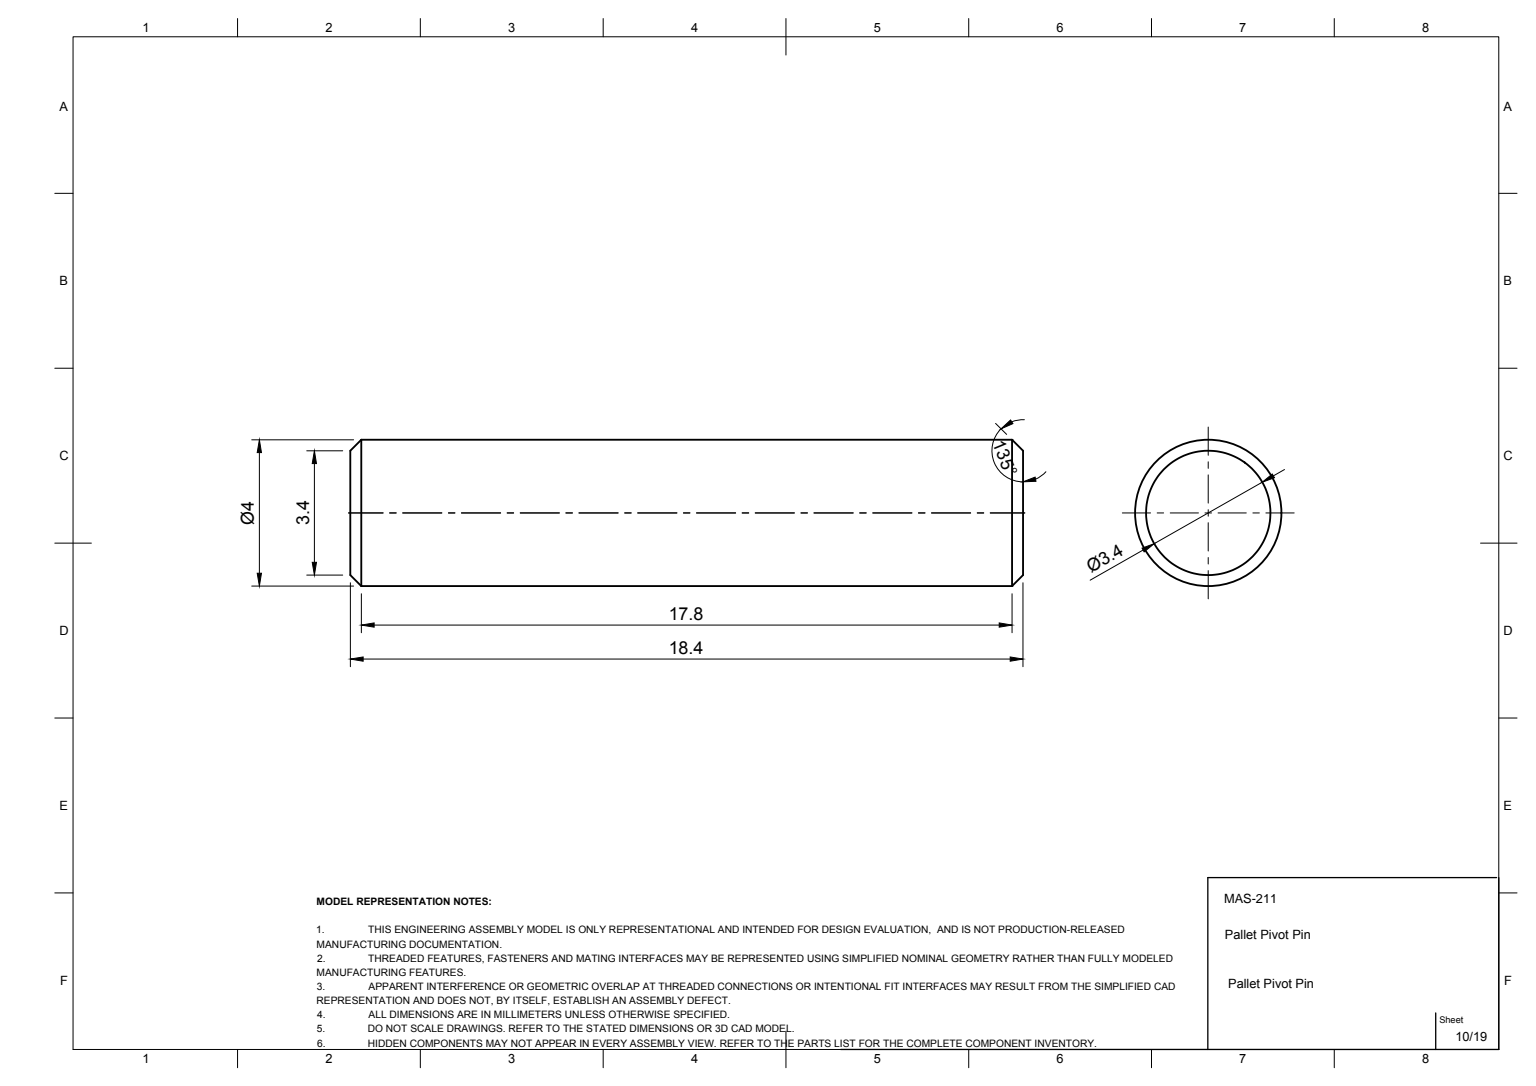
ISO-10303-21;
HEADER;
FILE_DESCRIPTION(
 (''),
 '2;1');
FILE_NAME ( 'Pallet Pivot Pin.step', '2026-10-05T20:07:59+06:00', ( '' ), ( '' ), 'STEP AP214', 'Unspecified', '' );
FILE_SCHEMA (('AUTOMOTIVE_DESIGN { 1 0 10303 214 3 1 1 }'));
ENDSEC;
DATA;
#10=MECHANICAL_DESIGN_GEOMETRIC_PRESENTATION_REPRESENTATION('',(#327),#196741);
#327=STYLED_ITEM('',(#196765),#346) ;
#346=MANIFOLD_SOLID_BREP('Pallet Pivot Pin',#8723) ;
#389=PLANE('',#8938) ;
#390=PLANE('',#8939) ;
#687=CIRCLE('',#8936,2.00000000000002) ;
#688=CIRCLE('',#8937,2.00000000000002) ;
#857=B_SPLINE_SURFACE_WITH_KNOTS('',1,3,((#113835,#113836,#113837,#113838,
#113839,#113840,#113841,#113842,#113843,#113844,#113845,#113846,#113847,
#113848,#113849,#113850,#113851,#113852,#113853),(#113854,#113855,#113856,
#113857,#113858,#113859,#113860,#113861,#113862,#113863,#113864,#113865,
#113866,#113867,#113868,#113869,#113870,#113871,#113872)),.UNSPECIFIED.,
 .F.,.T.,.F.,(2,2),(4,1,1,1,1,1,1,1,1,1,1,1,1,1,1,1,4),(0.,0.431146952730274),
(0.,0.667571568814079,1.33514313762816,2.00271471386765,2.67028629010715,
3.33785785892125,4.00542942773535,4.67300100397484,5.34057258021434,6.00814415645112,
6.67571573268789,7.34328730150198,8.01085887031606,8.67843044655556,9.34600202279505,
10.0135735916092,10.6811451604233),.UNSPECIFIED.) ;
#858=B_SPLINE_SURFACE_WITH_KNOTS('',3,1,((#113874,#113875),(#113876,#113877),
(#113878,#113879),(#113880,#113881),(#113882,#113883),(#113884,#113885),
(#113886,#113887),(#113888,#113889),(#113890,#113891),(#113892,#113893),
(#113894,#113895),(#113896,#113897),(#113898,#113899),(#113900,#113901),
(#113902,#113903),(#113904,#113905),(#113906,#113907),(#113908,#113909),
(#113910,#113911)),.UNSPECIFIED.,.T.,.F.,.F.,(4,1,1,1,1,1,1,1,1,1,1,1,1,
1,1,1,4),(2,2),(0.,0.667571568814083,1.33514313762817,2.00271471386766,
2.67028629010715,3.33785785892125,4.00542942773535,4.67300100397484,5.34057258021433,
6.00814415645111,6.67571573268789,7.34328730150198,8.01085887031607,8.67843044655557,
9.34600202279507,10.0135735916092,10.6811451604233),(0.,0.431146952730387),
 .UNSPECIFIED.) ;
#1009=FACE_OUTER_BOUND('',#1514,.T.) ;
#1010=FACE_OUTER_BOUND('',#1515,.T.) ;
#1011=FACE_OUTER_BOUND('',#1516,.T.) ;
#1012=FACE_OUTER_BOUND('',#1517,.T.) ;
#1013=FACE_OUTER_BOUND('',#1518,.T.) ;
#1514=EDGE_LOOP('',(#6350,#6351,#6352,#6353)) ;
#1515=EDGE_LOOP('',(#6354)) ;
#1516=EDGE_LOOP('',(#6355)) ;
#1517=EDGE_LOOP('',(#6356,#6357,#6358,#6359)) ;
#1518=EDGE_LOOP('',(#6360,#6361,#6362,#6363)) ;
#2007=LINE('',#113791,#2710) ;
#2008=LINE('',#113873,#2711) ;
#2009=LINE('',#113912,#2712) ;
#2710=VECTOR('',#9981,2.00000000000003) ;
#2711=VECTOR('',#9988,10.) ;
#2712=VECTOR('',#9989,10.) ;
#3433=B_SPLINE_CURVE_WITH_KNOTS('',3,(#113795,#113796,#113797,#113798,#113799,
#113800,#113801,#113802,#113803,#113804,#113805,#113806,#113807,#113808,
#113809,#113810,#113811,#113812,#113813),.UNSPECIFIED.,.T.,.F.,(4,1,1,1,
1,1,1,1,1,1,1,1,1,1,1,1,4),(0.,0.667571568814079,1.33514313762816,2.00271471386765,
2.67028629010715,3.33785785892125,4.00542942773535,4.67300100397484,5.34057258021434,
6.00814415645112,6.67571573268789,7.34328730150198,8.01085887031606,8.67843044655556,
9.34600202279505,10.0135735916092,10.6811451604233),.UNSPECIFIED.) ;
#3434=B_SPLINE_CURVE_WITH_KNOTS('',3,(#113816,#113817,#113818,#113819,#113820,
#113821,#113822,#113823,#113824,#113825,#113826,#113827,#113828,#113829,
#113830,#113831,#113832,#113833,#113834),.UNSPECIFIED.,.T.,.F.,(4,1,1,1,
1,1,1,1,1,1,1,1,1,1,1,1,4),(0.,0.667571568814083,1.33514313762817,2.00271471386766,
2.67028629010715,3.33785785892125,4.00542942773535,4.67300100397484,5.34057258021433,
6.00814415645111,6.67571573268789,7.34328730150198,8.01085887031607,8.67843044655557,
9.34600202279507,10.0135735916092,10.6811451604233),.UNSPECIFIED.) ;
#3704=VERTEX_POINT('',#113788) ;
#3705=VERTEX_POINT('',#113790) ;
#3706=VERTEX_POINT('',#113794) ;
#3707=VERTEX_POINT('',#113815) ;
#4683=EDGE_CURVE('',#3704,#3704,#687,.T.) ;
#4684=EDGE_CURVE('',#3704,#3705,#2007,.T.) ;
#4685=EDGE_CURVE('',#3705,#3705,#688,.T.) ;
#4686=EDGE_CURVE('',#3706,#3706,#3433,.T.) ;
#4687=EDGE_CURVE('',#3707,#3707,#3434,.T.) ;
#4688=EDGE_CURVE('',#3704,#3706,#2008,.T.) ;
#4689=EDGE_CURVE('',#3705,#3707,#2009,.T.) ;
#6350=ORIENTED_EDGE('',*,*,#4683,.T.) ;
#6351=ORIENTED_EDGE('',*,*,#4684,.T.) ;
#6352=ORIENTED_EDGE('',*,*,#4685,.F.) ;
#6353=ORIENTED_EDGE('',*,*,#4684,.F.) ;
#6354=ORIENTED_EDGE('',*,*,#4686,.F.) ;
#6355=ORIENTED_EDGE('',*,*,#4687,.T.) ;
#6356=ORIENTED_EDGE('',*,*,#4688,.T.) ;
#6357=ORIENTED_EDGE('',*,*,#4686,.T.) ;
#6358=ORIENTED_EDGE('',*,*,#4688,.F.) ;
#6359=ORIENTED_EDGE('',*,*,#4683,.F.) ;
#6360=ORIENTED_EDGE('',*,*,#4685,.T.) ;
#6361=ORIENTED_EDGE('',*,*,#4689,.T.) ;
#6362=ORIENTED_EDGE('',*,*,#4687,.F.) ;
#6363=ORIENTED_EDGE('',*,*,#4689,.F.) ;
#8184=CYLINDRICAL_SURFACE('',#8935,2.00000000000003) ;
#8392=ADVANCED_FACE('',(#1009),#8184,.T.) ;
#8393=ADVANCED_FACE('',(#1010),#389,.T.) ;
#8394=ADVANCED_FACE('',(#1011),#390,.T.) ;
#8395=ADVANCED_FACE('',(#1012),#857,.T.) ;
#8396=ADVANCED_FACE('',(#1013),#858,.T.) ;
#8723=CLOSED_SHELL('',(#8392,#8393,#8394,#8395,#8396)) ;
#8935=AXIS2_PLACEMENT_3D('',#113787,#9977,#9978) ;
#8936=AXIS2_PLACEMENT_3D('',#113789,#9979,#9980) ;
#8937=AXIS2_PLACEMENT_3D('',#113792,#9982,#9983) ;
#8938=AXIS2_PLACEMENT_3D('',#113793,#9984,#9985) ;
#8939=AXIS2_PLACEMENT_3D('',#113814,#9986,#9987) ;
#9977=DIRECTION('center_axis',(0.,-1.,0.)) ;
#9978=DIRECTION('ref_axis',(0.587391769794684,0.,-0.809302729995068)) ;
#9979=DIRECTION('center_axis',(-6.57177564856263E-16,1.,-6.46151479728032E-16)) ;
#9980=DIRECTION('ref_axis',(-0.948327476740895,-5.55111512312572E-16,0.317293234813235)) ;
#9981=DIRECTION('',(0.,1.,0.)) ;
#9982=DIRECTION('center_axis',(1.11571400579693E-15,1.,3.09771438098241E-16)) ;
#9983=DIRECTION('ref_axis',(-0.948327476740895,1.11022302462514E-15,0.317293234813235)) ;
#9984=DIRECTION('center_axis',(0.,-1.,0.)) ;
#9985=DIRECTION('ref_axis',(0.,0.,-1.)) ;
#9986=DIRECTION('center_axis',(0.,1.,0.)) ;
#9987=DIRECTION('ref_axis',(0.,0.,1.)) ;
#9988=DIRECTION('',(0.415348703634992,-0.707106781186545,-0.572263448412299)) ;
#9989=DIRECTION('',(0.415348703634974,0.707106781186551,-0.572263448412304)) ;
#113787=CARTESIAN_POINT('Origin',(-28.8703041205685,-9.2000000000496,120.173187866852)) ;
#113788=CARTESIAN_POINT('',(-30.0450876601579,-8.90000000004959,121.791793326842)) ;
#113789=CARTESIAN_POINT('Origin',(-28.8703041205685,-8.90000000004959,120.173187866852)) ;
#113790=CARTESIAN_POINT('',(-30.0450876601579,8.90000000004959,121.791793326842)) ;
#113791=CARTESIAN_POINT('',(-30.0450876601579,-9.2000000000496,121.791793326842)) ;
#113792=CARTESIAN_POINT('Origin',(-28.8703041205685,8.90000000004959,120.173187866852)) ;
#113793=CARTESIAN_POINT('Origin',(-30.0450876601579,-9.2000000000496,121.791793326842)) ;
#113794=CARTESIAN_POINT('',(-29.8688701292195,-9.2000000000496,121.549002507844)) ;
#113795=CARTESIAN_POINT('Ctrl Pts',(-29.8688701292195,-9.2000000000496,
121.549002507844)) ;
#113796=CARTESIAN_POINT('Ctrl Pts',(-29.6888722586779,-9.2000000000496,
121.679801257268)) ;
#113797=CARTESIAN_POINT('Ctrl Pts',(-29.2766671363574,-9.2000000000496,
121.869462570365)) ;
#113798=CARTESIAN_POINT('Ctrl Pts',(-28.5966094899589,-9.20000000004961,
121.895918474133)) ;
#113799=CARTESIAN_POINT('Ctrl Pts',(-27.9581738536376,-9.20000000004958,
121.660008974116)) ;
#113800=CARTESIAN_POINT('Ctrl Pts',(-27.4586313028868,-9.20000000004961,
121.197792875516)) ;
#113801=CARTESIAN_POINT('Ctrl Pts',(-27.1739845654614,-9.20000000004959,
120.579569231899)) ;
#113802=CARTESIAN_POINT('Ctrl Pts',(-27.1475967294287,-9.2000000000496,
119.899485204542)) ;
#113803=CARTESIAN_POINT('Ctrl Pts',(-27.3834704179729,-9.20000000004961,
119.261061767752)) ;
#113804=CARTESIAN_POINT('Ctrl Pts',(-27.8457060572027,-9.20000000004959,
118.761512772263)) ;
#113805=CARTESIAN_POINT('Ctrl Pts',(-28.4639187630298,-9.20000000004959,
118.476869616603)) ;
#113806=CARTESIAN_POINT('Ctrl Pts',(-29.1440090539224,-9.2000000000496,
118.450479738512)) ;
#113807=CARTESIAN_POINT('Ctrl Pts',(-29.7824289744744,-9.20000000004958,
118.686354577768)) ;
#113808=CARTESIAN_POINT('Ctrl Pts',(-30.2819799090915,-9.2000000000496,
119.148589579807)) ;
#113809=CARTESIAN_POINT('Ctrl Pts',(-30.5666217872644,-9.2000000000496,
119.766803935434)) ;
#113810=CARTESIAN_POINT('Ctrl Pts',(-30.593025972774,-9.20000000004959,
120.446909151552)) ;
#113811=CARTESIAN_POINT('Ctrl Pts',(-30.3571041737437,-9.2000000000496,
121.085287178393)) ;
#113812=CARTESIAN_POINT('Ctrl Pts',(-30.0490282665823,-9.20000000004959,
121.418401787627)) ;
#113813=CARTESIAN_POINT('Ctrl Pts',(-29.8688701292195,-9.2000000000496,
121.549002507844)) ;
#113814=CARTESIAN_POINT('Origin',(-30.0450876601579,9.2000000000496,121.791793326842)) ;
#113815=CARTESIAN_POINT('',(-29.8688701292195,9.2000000000496,121.549002507844)) ;
#113816=CARTESIAN_POINT('Ctrl Pts',(-29.8688701292195,9.2000000000496,121.549002507844)) ;
#113817=CARTESIAN_POINT('Ctrl Pts',(-29.6888722586779,9.2000000000496,121.679801257268)) ;
#113818=CARTESIAN_POINT('Ctrl Pts',(-29.2766671363573,9.20000000004959,
121.869462570365)) ;
#113819=CARTESIAN_POINT('Ctrl Pts',(-28.5966094899589,9.20000000004961,
121.895918474133)) ;
#113820=CARTESIAN_POINT('Ctrl Pts',(-27.9581738536375,9.20000000004957,
121.660008974116)) ;
#113821=CARTESIAN_POINT('Ctrl Pts',(-27.4586313028868,9.20000000004962,
121.197792875516)) ;
#113822=CARTESIAN_POINT('Ctrl Pts',(-27.1739845654613,9.20000000004957,
120.579569231898)) ;
#113823=CARTESIAN_POINT('Ctrl Pts',(-27.1475967294288,9.20000000004963,
119.899485204542)) ;
#113824=CARTESIAN_POINT('Ctrl Pts',(-27.3834704179728,9.20000000004958,
119.261061767752)) ;
#113825=CARTESIAN_POINT('Ctrl Pts',(-27.8457060572028,9.2000000000496,118.761512772263)) ;
#113826=CARTESIAN_POINT('Ctrl Pts',(-28.4639187630298,9.20000000004957,
118.476869616603)) ;
#113827=CARTESIAN_POINT('Ctrl Pts',(-29.1440090539225,9.20000000004963,
118.450479738513)) ;
#113828=CARTESIAN_POINT('Ctrl Pts',(-29.7824289744743,9.20000000004957,
118.686354577768)) ;
#113829=CARTESIAN_POINT('Ctrl Pts',(-30.2819799090916,9.2000000000496,119.148589579807)) ;
#113830=CARTESIAN_POINT('Ctrl Pts',(-30.5666217872643,9.2000000000496,119.766803935434)) ;
#113831=CARTESIAN_POINT('Ctrl Pts',(-30.593025972774,9.20000000004959,120.446909151552)) ;
#113832=CARTESIAN_POINT('Ctrl Pts',(-30.3571041737438,9.2000000000496,121.085287178393)) ;
#113833=CARTESIAN_POINT('Ctrl Pts',(-30.0490282665823,9.2000000000496,121.418401787627)) ;
#113834=CARTESIAN_POINT('Ctrl Pts',(-29.8688701292195,9.2000000000496,121.549002507844)) ;
#113835=CARTESIAN_POINT('Ctrl Pts',(-30.0450876601579,-8.90000000004959,
121.791793326842)) ;
#113836=CARTESIAN_POINT('Ctrl Pts',(-29.8333254600702,-8.90000000004959,
121.945674208536)) ;
#113837=CARTESIAN_POINT('Ctrl Pts',(-29.3483782557085,-8.9000000000496,
122.168805164942)) ;
#113838=CARTESIAN_POINT('Ctrl Pts',(-28.548310438228,-8.90000000004961,
122.199929757708)) ;
#113839=CARTESIAN_POINT('Ctrl Pts',(-27.7972096887258,-8.90000000004958,
121.922389169964)) ;
#113840=CARTESIAN_POINT('Ctrl Pts',(-27.2095125702208,-8.9000000000496,
121.378605523632)) ;
#113841=CARTESIAN_POINT('Ctrl Pts',(-26.8746340558794,-8.90000000004959,
120.651283590262)) ;
#113842=CARTESIAN_POINT('Ctrl Pts',(-26.8435895428338,-8.90000000004959,
119.851184734958)) ;
#113843=CARTESIAN_POINT('Ctrl Pts',(-27.1210879996609,-8.90000000004961,
119.100098338637)) ;
#113844=CARTESIAN_POINT('Ctrl Pts',(-27.6648946349492,-8.90000000004958,
118.512393637684)) ;
#113845=CARTESIAN_POINT('Ctrl Pts',(-28.3922036993925,-8.90000000004959,
118.177519337191)) ;
#113846=CARTESIAN_POINT('Ctrl Pts',(-29.1923099252244,-8.9000000000496,
118.146472421837)) ;
#113847=CARTESIAN_POINT('Ctrl Pts',(-29.9433921833963,-8.90000000004959,
118.423972232679)) ;
#113848=CARTESIAN_POINT('Ctrl Pts',(-30.5310991659206,-8.90000000004959,
118.967778117292)) ;
#113849=CARTESIAN_POINT('Ctrl Pts',(-30.8659719637261,-8.90000000004961,
119.695089123834)) ;
#113850=CARTESIAN_POINT('Ctrl Pts',(-30.8970357112146,-8.90000000004959,
120.495212908351)) ;
#113851=CARTESIAN_POINT('Ctrl Pts',(-30.619480653913,-8.9000000000496,121.246245879451)) ;
#113852=CARTESIAN_POINT('Ctrl Pts',(-30.2570384098916,-8.90000000004959,
121.63814542126)) ;
#113853=CARTESIAN_POINT('Ctrl Pts',(-30.0450876601579,-8.90000000004959,
121.791793326842)) ;
#113854=CARTESIAN_POINT('Ctrl Pts',(-29.8688701292195,-9.2000000000496,
121.549002507844)) ;
#113855=CARTESIAN_POINT('Ctrl Pts',(-29.6888722586779,-9.2000000000496,
121.679801257268)) ;
#113856=CARTESIAN_POINT('Ctrl Pts',(-29.2766671363574,-9.2000000000496,
121.869462570365)) ;
#113857=CARTESIAN_POINT('Ctrl Pts',(-28.5966094899589,-9.20000000004961,
121.895918474133)) ;
#113858=CARTESIAN_POINT('Ctrl Pts',(-27.9581738536376,-9.20000000004958,
121.660008974116)) ;
#113859=CARTESIAN_POINT('Ctrl Pts',(-27.4586313028868,-9.20000000004961,
121.197792875516)) ;
#113860=CARTESIAN_POINT('Ctrl Pts',(-27.1739845654614,-9.20000000004959,
120.579569231899)) ;
#113861=CARTESIAN_POINT('Ctrl Pts',(-27.1475967294287,-9.2000000000496,
119.899485204542)) ;
#113862=CARTESIAN_POINT('Ctrl Pts',(-27.3834704179729,-9.20000000004961,
119.261061767752)) ;
#113863=CARTESIAN_POINT('Ctrl Pts',(-27.8457060572027,-9.20000000004959,
118.761512772263)) ;
#113864=CARTESIAN_POINT('Ctrl Pts',(-28.4639187630298,-9.20000000004959,
118.476869616603)) ;
#113865=CARTESIAN_POINT('Ctrl Pts',(-29.1440090539224,-9.2000000000496,
118.450479738512)) ;
#113866=CARTESIAN_POINT('Ctrl Pts',(-29.7824289744744,-9.20000000004958,
118.686354577768)) ;
#113867=CARTESIAN_POINT('Ctrl Pts',(-30.2819799090915,-9.2000000000496,
119.148589579807)) ;
#113868=CARTESIAN_POINT('Ctrl Pts',(-30.5666217872644,-9.2000000000496,
119.766803935434)) ;
#113869=CARTESIAN_POINT('Ctrl Pts',(-30.593025972774,-9.20000000004959,
120.446909151552)) ;
#113870=CARTESIAN_POINT('Ctrl Pts',(-30.3571041737437,-9.2000000000496,
121.085287178393)) ;
#113871=CARTESIAN_POINT('Ctrl Pts',(-30.0490282665823,-9.20000000004959,
121.418401787627)) ;
#113872=CARTESIAN_POINT('Ctrl Pts',(-29.8688701292195,-9.2000000000496,
121.549002507844)) ;
#113873=CARTESIAN_POINT('',(-30.0450876601579,-8.90000000004959,121.791793326842)) ;
#113874=CARTESIAN_POINT('Ctrl Pts',(-30.0450876601579,8.90000000004959,
121.791793326842)) ;
#113875=CARTESIAN_POINT('Ctrl Pts',(-29.8688701292195,9.2000000000496,121.549002507844)) ;
#113876=CARTESIAN_POINT('Ctrl Pts',(-29.8333254600701,8.9000000000496,121.945674208536)) ;
#113877=CARTESIAN_POINT('Ctrl Pts',(-29.6888722586779,9.2000000000496,121.679801257268)) ;
#113878=CARTESIAN_POINT('Ctrl Pts',(-29.3483782557084,8.90000000004959,
122.168805164942)) ;
#113879=CARTESIAN_POINT('Ctrl Pts',(-29.2766671363573,9.20000000004959,
121.869462570365)) ;
#113880=CARTESIAN_POINT('Ctrl Pts',(-28.548310438228,8.90000000004961,122.199929757709)) ;
#113881=CARTESIAN_POINT('Ctrl Pts',(-28.5966094899589,9.20000000004961,
121.895918474133)) ;
#113882=CARTESIAN_POINT('Ctrl Pts',(-27.7972096887257,8.90000000004957,
121.922389169964)) ;
#113883=CARTESIAN_POINT('Ctrl Pts',(-27.9581738536375,9.20000000004957,
121.660008974116)) ;
#113884=CARTESIAN_POINT('Ctrl Pts',(-27.2095125702209,8.90000000004962,
121.378605523633)) ;
#113885=CARTESIAN_POINT('Ctrl Pts',(-27.4586313028868,9.20000000004962,
121.197792875516)) ;
#113886=CARTESIAN_POINT('Ctrl Pts',(-26.8746340558793,8.90000000004957,
120.651283590261)) ;
#113887=CARTESIAN_POINT('Ctrl Pts',(-27.1739845654613,9.20000000004957,
120.579569231898)) ;
#113888=CARTESIAN_POINT('Ctrl Pts',(-26.8435895428339,8.90000000004962,
119.851184734958)) ;
#113889=CARTESIAN_POINT('Ctrl Pts',(-27.1475967294288,9.20000000004963,
119.899485204542)) ;
#113890=CARTESIAN_POINT('Ctrl Pts',(-27.1210879996608,8.90000000004958,
119.100098338637)) ;
#113891=CARTESIAN_POINT('Ctrl Pts',(-27.3834704179728,9.20000000004958,
119.261061767752)) ;
#113892=CARTESIAN_POINT('Ctrl Pts',(-27.6648946349493,8.9000000000496,118.512393637685)) ;
#113893=CARTESIAN_POINT('Ctrl Pts',(-27.8457060572028,9.2000000000496,118.761512772263)) ;
#113894=CARTESIAN_POINT('Ctrl Pts',(-28.3922036993924,8.90000000004957,
118.177519337191)) ;
#113895=CARTESIAN_POINT('Ctrl Pts',(-28.4639187630298,9.20000000004957,
118.476869616603)) ;
#113896=CARTESIAN_POINT('Ctrl Pts',(-29.1923099252245,8.90000000004963,
118.146472421837)) ;
#113897=CARTESIAN_POINT('Ctrl Pts',(-29.1440090539225,9.20000000004963,
118.450479738513)) ;
#113898=CARTESIAN_POINT('Ctrl Pts',(-29.9433921833963,8.90000000004956,
118.423972232679)) ;
#113899=CARTESIAN_POINT('Ctrl Pts',(-29.7824289744743,9.20000000004957,
118.686354577768)) ;
#113900=CARTESIAN_POINT('Ctrl Pts',(-30.5310991659207,8.90000000004961,
118.967778117292)) ;
#113901=CARTESIAN_POINT('Ctrl Pts',(-30.2819799090916,9.2000000000496,119.148589579807)) ;
#113902=CARTESIAN_POINT('Ctrl Pts',(-30.8659719637261,8.90000000004959,
119.695089123834)) ;
#113903=CARTESIAN_POINT('Ctrl Pts',(-30.5666217872643,9.2000000000496,119.766803935434)) ;
#113904=CARTESIAN_POINT('Ctrl Pts',(-30.8970357112146,8.90000000004959,
120.495212908351)) ;
#113905=CARTESIAN_POINT('Ctrl Pts',(-30.593025972774,9.20000000004959,120.446909151552)) ;
#113906=CARTESIAN_POINT('Ctrl Pts',(-30.619480653913,8.9000000000496,121.246245879451)) ;
#113907=CARTESIAN_POINT('Ctrl Pts',(-30.3571041737438,9.2000000000496,121.085287178393)) ;
#113908=CARTESIAN_POINT('Ctrl Pts',(-30.2570384098916,8.90000000004959,
121.63814542126)) ;
#113909=CARTESIAN_POINT('Ctrl Pts',(-30.0490282665823,9.2000000000496,121.418401787627)) ;
#113910=CARTESIAN_POINT('Ctrl Pts',(-30.0450876601579,8.90000000004959,
121.791793326842)) ;
#113911=CARTESIAN_POINT('Ctrl Pts',(-29.8688701292195,9.2000000000496,121.549002507844)) ;
#113912=CARTESIAN_POINT('',(-30.0450876601579,8.90000000004959,121.791793326842)) ;
#196737=UNCERTAINTY_MEASURE_WITH_UNIT(LENGTH_MEASURE(0.01),#196742,
'DISTANCE_ACCURACY_VALUE',
'Maximum model space distance between geometric entities at asserted c
onnectivities') ;
#196738=UNCERTAINTY_MEASURE_WITH_UNIT(LENGTH_MEASURE(0.01),#196742,
'DISTANCE_ACCURACY_VALUE',
'Maximum model space distance between geometric entities at asserted c
onnectivities') ;
#196740=(
GEOMETRIC_REPRESENTATION_CONTEXT(3)
GLOBAL_UNCERTAINTY_ASSIGNED_CONTEXT((#196737))
GLOBAL_UNIT_ASSIGNED_CONTEXT((#196742,#196744,#196745))
REPRESENTATION_CONTEXT('','3D')
) ;
#196741=(
GEOMETRIC_REPRESENTATION_CONTEXT(3)
GLOBAL_UNCERTAINTY_ASSIGNED_CONTEXT((#196738))
GLOBAL_UNIT_ASSIGNED_CONTEXT((#196742,#196744,#196745))
REPRESENTATION_CONTEXT('','3D')
) ;
#196742=(
LENGTH_UNIT()
NAMED_UNIT(*)
SI_UNIT(.MILLI.,.METRE.)
) ;
#196744=(
NAMED_UNIT(*)
PLANE_ANGLE_UNIT()
SI_UNIT($,.RADIAN.)
) ;
#196745=(
NAMED_UNIT(*)
SI_UNIT($,.STERADIAN.)
SOLID_ANGLE_UNIT()
) ;
#196753=PRODUCT_DEFINITION_CONTEXT('part definition',#196761,'design') ;
#196761=APPLICATION_CONTEXT(
'Core Data for Automotive Mechanical Design Process') ;
#196762=PRODUCT_CONTEXT('part definition',#196761,'mechanical') ;
#196765=PRESENTATION_STYLE_ASSIGNMENT((#196767)) ;
#196767=SURFACE_STYLE_USAGE(.BOTH.,#196769) ;
#196769=SURFACE_SIDE_STYLE('',(#196771)) ;
#196771=SURFACE_STYLE_FILL_AREA(#196773) ;
#196773=FILL_AREA_STYLE('Steel - Satin',(#196775)) ;
#196775=FILL_AREA_STYLE_COLOUR('Steel - Satin',#196777) ;
#196777=COLOUR_RGB('Steel - Satin', 0.09019608, 0.27058824, 0.51372549) ;
#196971=CARTESIAN_POINT ( '', ( 0.0, 0.0, 0.0 ) ) ;
#196972=DIRECTION ( '', ( 0.0, 0.0, 1.0 ) ) ;
#196973=DIRECTION ( '', ( 1.0, 0.0, 0.0 ) ) ;
#196974=AXIS2_PLACEMENT_3D ( '', #196971, #196972, #196973 ) ;
#196975=ADVANCED_BREP_SHAPE_REPRESENTATION ( 'Pallet Pivot Pin', ( #346, #196974, #196985, #197342 ), #196740 ) ;
#196976=PRODUCT( 'Pallet Pivot Pin', 'Pallet Pivot Pin', '', ( #196762 ) ) ;
#196977=PRODUCT_DEFINITION_FORMATION ( '', '', #196976 ) ;
#196978=PRODUCT_DEFINITION( 'Pallet Pivot Pin', 'Pallet Pivot Pin', #196977, #196753 ) ;
#196979=PRODUCT_DEFINITION_SHAPE ( '', '', #196978 ) ;
#196980=SHAPE_DEFINITION_REPRESENTATION ( #196979, #196975 ) ;
#196982=CARTESIAN_POINT ( '', ( 0.0, 0.0, 0.0 ) ) ;
#196983=DIRECTION ( '', ( 0.0, 0.0, 1.0 ) ) ;
#196984=DIRECTION ( '', ( 1.0, 0.0, 0.0 ) ) ;
#196985=AXIS2_PLACEMENT_3D ( '', #196982, #196983, #196984 ) ;
#197339=CARTESIAN_POINT ( '', ( 0.0, 0.0, 0.0 ) ) ;
#197340=DIRECTION ( '', ( 0.0, 0.0, 1.0 ) ) ;
#197341=DIRECTION ( '', ( 1.0, 0.0, 0.0 ) ) ;
#197342=AXIS2_PLACEMENT_3D ( '', #197339, #197340, #197341 ) ;
ENDSEC;
END-ISO-10303-21;
